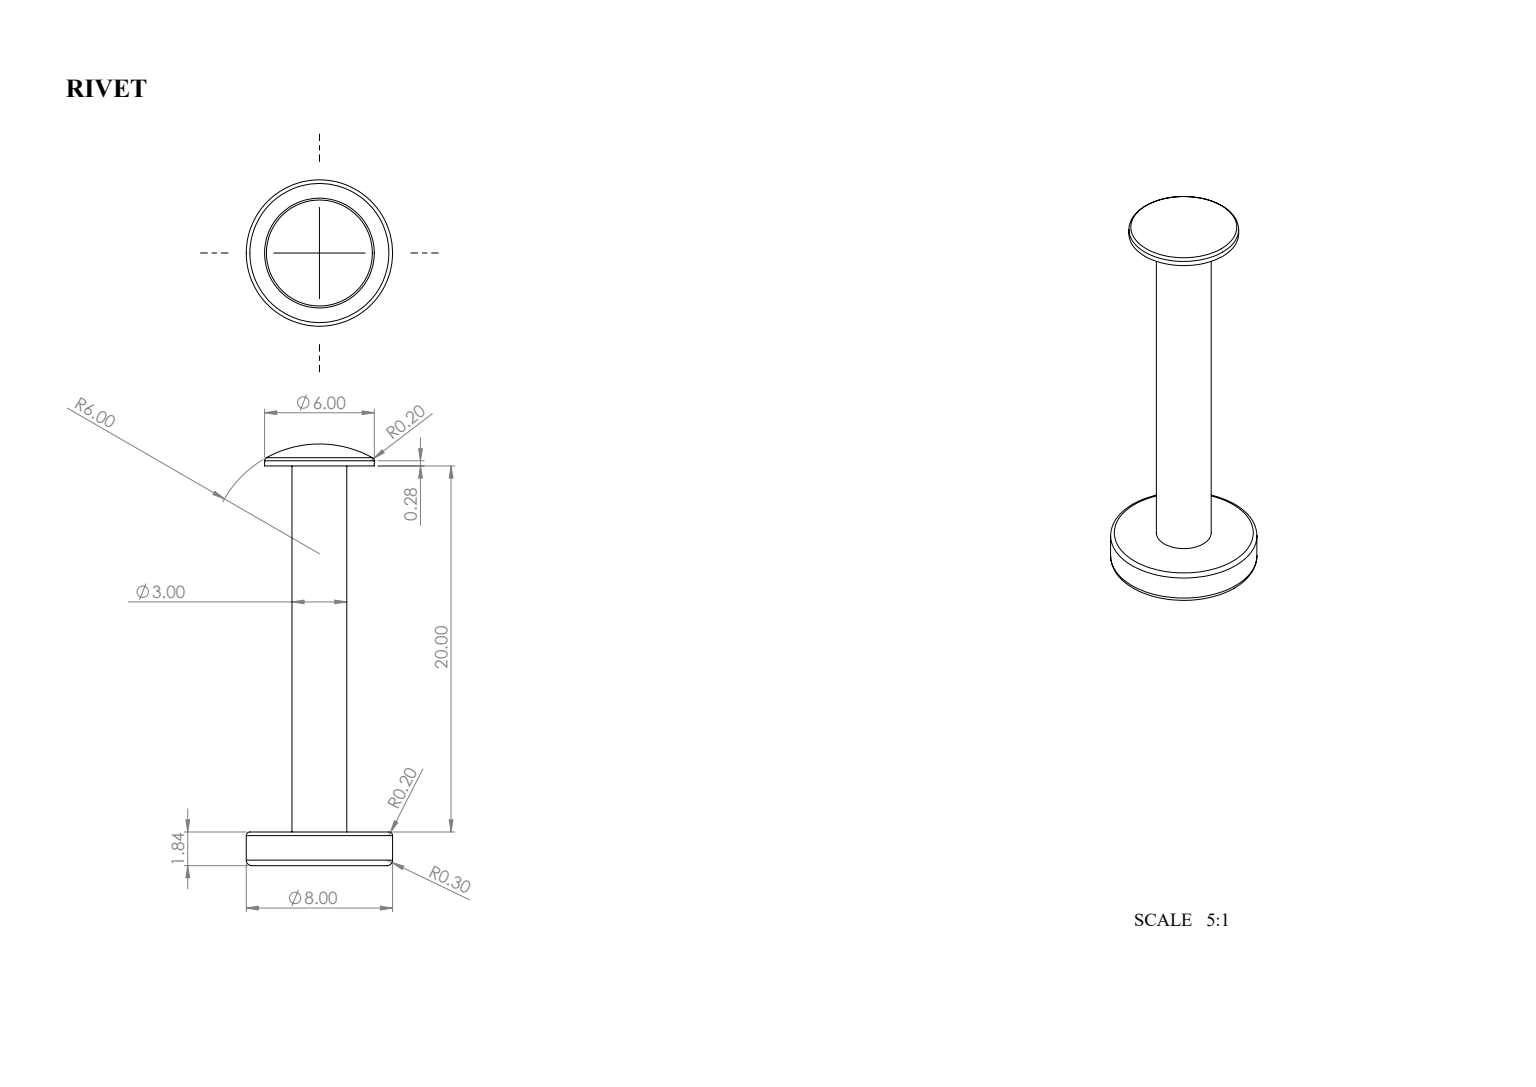
ISO-10303-21;
HEADER;
FILE_DESCRIPTION (('STEP AP214'),
    '1' );
FILE_NAME ('1.4 Rivet.step',
    '2026-10-07T05:30:18',
    ( '' ),
    ( '' ),
    'SwSTEP 2.0',
    'SolidWorks 2021',
    '' );
FILE_SCHEMA (( 'AUTOMOTIVE_DESIGN' ));
ENDSEC;

DATA;
#994=LINE ( 'NONE', #30968, #8060 ) ;
#1053=EDGE_CURVE ( 'NONE', #87334, #57215, #41639, .T. ) ;
#1123=FACE_OUTER_BOUND ( 'NONE', #83548, .T. ) ;
#1979=DIRECTION ( 'NONE',  ( 1.257568779154408793E-17, 1.000000000000000000, -0.000000000000000000 ) ) ;
#2099=EDGE_CURVE ( 'NONE', #84532, #89907, #23376, .T. ) ;
#2341=DIRECTION ( 'NONE',  ( 1.257568779154408793E-17, 1.000000000000000000, -0.000000000000000000 ) ) ;
#2551=DIRECTION ( 'NONE',  ( 1.224646799147353454E-16, -1.540077580099091832E-33, 1.000000000000000000 ) ) ;
#2715=VECTOR ( 'NONE', #9049, 1000.000000000000000 ) ;
#2831=CARTESIAN_POINT ( 'NONE',  ( -3.999999999999999112, 1.639999999999999014, 0.000000000000000000 ) ) ;
#2905=AXIS2_PLACEMENT_3D ( 'NONE', #26099, #87086, #58050 ) ;
#2964=CYLINDRICAL_SURFACE ( 'NONE', #23170, 3.000000000000000000 ) ;
#3145=CIRCLE ( 'NONE', #81349, 3.000000000000000000 ) ;
#3237=ORIENTED_EDGE ( 'NONE', *, *, #29922, .F. ) ;
#3507=ORIENTED_EDGE ( 'NONE', *, *, #71148, .T. ) ;
#3526=DIRECTION ( 'NONE',  ( 1.224646799147353207E-16, -1.540077580099091490E-33, 1.000000000000000000 ) ) ;
#3594=CARTESIAN_POINT ( 'NONE',  ( 2.781662917646512463E-16, 22.11937003968011695, 0.000000000000000000 ) ) ;
#3598=ORIENTED_EDGE ( 'NONE', *, *, #21717, .T. ) ;
#3600=AXIS2_PLACEMENT_3D ( 'NONE', #83921, #45930, #15451 ) ;
#3653=DIRECTION ( 'NONE',  ( -1.000000000000000000, 0.000000000000000000, 0.000000000000000000 ) ) ;
#3899=AXIS2_PLACEMENT_3D ( 'NONE', #71999, #3526, #32526 ) ;
#4516=UNCERTAINTY_MEASURE_WITH_UNIT (LENGTH_MEASURE( 1.000000000000000082E-05 ), #93288, 'distance_accuracy_value', 'NONE');
#4564=DIRECTION ( 'NONE',  ( 1.000000000000000000, 0.000000000000000000, 0.000000000000000000 ) ) ;
#4762=( LENGTH_UNIT ( ) NAMED_UNIT ( * ) SI_UNIT ( .MILLI., .METRE. ) );
#4915=ADVANCED_FACE ( 'NONE', ( #17323 ), #7942, .T. ) ;
#5067=ORIENTED_EDGE ( 'NONE', *, *, #61966, .F. ) ;
#5482=AXIS2_PLACEMENT_3D ( 'NONE', #73120, #20635, #81616 ) ;
#5598=ORIENTED_EDGE ( 'NONE', *, *, #25141, .F. ) ;
#5632=ORIENTED_EDGE ( 'NONE', *, *, #30715, .T. ) ;
#5880=ORIENTED_EDGE ( 'NONE', *, *, #27317, .T. ) ;
#6443=ORIENTED_EDGE ( 'NONE', *, *, #20709, .F. ) ;
#6533=( NAMED_UNIT ( * ) PLANE_ANGLE_UNIT ( ) SI_UNIT ( $, .RADIAN. ) );
#6537=EDGE_LOOP ( 'NONE', ( #7707, #54007, #79650, #25763 ) ) ;
#6599=CARTESIAN_POINT ( 'NONE',  ( 2.897438467171757030E-16, 23.03999999999999915, 0.000000000000000000 ) ) ;
#6634=ORIENTED_EDGE ( 'NONE', *, *, #41779, .F. ) ;
#6707=CARTESIAN_POINT ( 'NONE',  ( -3.999999999999999112, 23.03999999999999915, 0.000000000000000000 ) ) ;
#7105=AXIS2_PLACEMENT_3D ( 'NONE', #24931, #81354, #96380 ) ;
#7707=ORIENTED_EDGE ( 'NONE', *, *, #44953, .F. ) ;
#7942=TOROIDAL_SURFACE ( 'NONE', #95802, 3.699999999999999289, 0.2999999999999999889 ) ;
#8060=VECTOR ( 'NONE', #31455, 1000.000000000000000 ) ;
#8125=ORIENTED_EDGE ( 'NONE', *, *, #27988, .F. ) ;
#8242=DIRECTION ( 'NONE',  ( 1.257568779154408793E-17, 1.000000000000000000, -0.000000000000000000 ) ) ;
#8286=ORIENTED_EDGE ( 'NONE', *, *, #30815, .F. ) ;
#8311=CARTESIAN_POINT ( 'NONE',  ( 3.699999999999999289, -3.175805879500891925E-16, 0.000000000000000000 ) ) ;
#8356=DIRECTION ( 'NONE',  ( 1.000000000000000000, -1.257568779154408793E-17, 0.000000000000000000 ) ) ;
#8475=DIRECTION ( 'NONE',  ( -1.000000000000000000, 0.000000000000000000, 0.000000000000000000 ) ) ;
#8500=DIRECTION ( 'NONE',  ( 1.000000000000000000, -1.257568779154408793E-17, 0.000000000000000000 ) ) ;
#8588=CARTESIAN_POINT ( 'NONE',  ( 2.062412797813223616E-17, 1.639999999999999014, 0.000000000000000000 ) ) ;
#8590=DIRECTION ( 'NONE',  ( -1.224646799147353207E-16, 1.540077580099091490E-33, 1.000000000000000000 ) ) ;
#9030=ORIENTED_EDGE ( 'NONE', *, *, #22024, .T. ) ;
#9049=DIRECTION ( 'NONE',  ( 1.257568779154408793E-17, 1.000000000000000000, -0.000000000000000000 ) ) ;
#9309=SURFACE_STYLE_FILL_AREA ( #54796 ) ;
#9311=ADVANCED_FACE ( 'NONE', ( #80057 ), #12052, .T. ) ;
#9416=FACE_BOUND ( 'NONE', #37266, .T. ) ;
#9569=DIRECTION ( 'NONE',  ( -1.257568779154408793E-17, -1.000000000000000000, 0.000000000000000000 ) ) ;
#10064=ADVANCED_FACE ( 'NONE', ( #86449 ), #2964, .T. ) ;
#10245=EDGE_LOOP ( 'NONE', ( #5632, #31028 ) ) ;
#10593=FILL_AREA_STYLE_COLOUR ( '', #94402 ) ;
#10723=CIRCLE ( 'NONE', #42697, 3.799999999999998934 ) ;
#10781=FILL_AREA_STYLE ('',( #92794 ) ) ;
#10794=DIRECTION ( 'NONE',  ( 1.000000000000000000, -1.257568779154408793E-17, 0.000000000000000000 ) ) ;
#10894=DIRECTION ( 'NONE',  ( -1.000000000000000000, 1.257568779154408793E-17, 0.000000000000000000 ) ) ;
#11328=CIRCLE ( 'NONE', #49632, 5.999999999999998224 ) ;
#11443=CARTESIAN_POINT ( 'NONE',  ( 2.746530213673227803E-16, 21.83999999999999986, 0.000000000000000000 ) ) ;
#11508=CARTESIAN_POINT ( 'NONE',  ( -2.999999999999999556, 22.11937003968011695, 0.000000000000000000 ) ) ;
#11523=EDGE_CURVE ( 'NONE', #83267, #75676, #84199, .T. ) ;
#11994=VERTEX_POINT ( 'NONE', #72205 ) ;
#12052=CYLINDRICAL_SURFACE ( 'NONE', #51536, 3.999999999999999112 ) ;
#12174=ORIENTED_EDGE ( 'NONE', *, *, #68028, .F. ) ;
#12439=DIRECTION ( 'NONE',  ( 1.257568779154408793E-17, 1.000000000000000000, -0.000000000000000000 ) ) ;
#12451=CARTESIAN_POINT ( 'NONE',  ( 7.347880794884118750E-16, 17.03999999999999915, 0.000000000000000000 ) ) ;
#12652=VERTEX_POINT ( 'NONE', #39645 ) ;
#12891=AXIS2_PLACEMENT_3D ( 'NONE', #27041, #42546, #4564 ) ;
#13685=CARTESIAN_POINT ( 'NONE',  ( -3.799999999999998934, 1.839999999999999636, 0.000000000000000000 ) ) ;
#13872=EDGE_LOOP ( 'NONE', ( #80023, #45997, #3507, #3237 ) ) ;
#14332=CARTESIAN_POINT ( 'NONE',  ( 2.746530213673227803E-16, 21.83999999999999986, 0.000000000000000000 ) ) ;
#14481=UNCERTAINTY_MEASURE_WITH_UNIT (LENGTH_MEASURE( 1.000000000000000082E-05 ), #4762, 'distance_accuracy_value', 'NONE');
#14523=AXIS2_PLACEMENT_3D ( 'NONE', #8588, #9569, #70081 ) ;
#14902=DIRECTION ( 'NONE',  ( 1.257568779154408793E-17, 1.000000000000000000, -0.000000000000000000 ) ) ;
#15052=CARTESIAN_POINT ( 'NONE',  ( -1.499999999999998668, 1.840000000000001412, 0.000000000000000000 ) ) ;
#15404=EDGE_CURVE ( 'NONE', #57215, #87334, #18798, .T. ) ;
#15451=DIRECTION ( 'NONE',  ( -1.000000000000000000, 0.000000000000000000, 0.000000000000000000 ) ) ;
#15628=DIRECTION ( 'NONE',  ( 0.000000000000000000, -0.000000000000000000, -1.000000000000000000 ) ) ;
#15653=VERTEX_POINT ( 'NONE', #15052 ) ;
#15929=STYLED_ITEM ( 'NONE', ( #47796 ), #4915 ) ;
#16369=EDGE_CURVE ( 'NONE', #44561, #15653, #23678, .T. ) ;
#16487=ORIENTED_EDGE ( 'NONE', *, *, #71397, .T. ) ;
#16857=CARTESIAN_POINT ( 'NONE',  ( 2.313926553644105868E-17, 1.839999999999999636, 0.000000000000000000 ) ) ;
#17128=CIRCLE ( 'NONE', #21912, 3.000000000000000000 ) ;
#17130=ORIENTED_EDGE ( 'NONE', *, *, #2099, .F. ) ;
#17323=FACE_OUTER_BOUND ( 'NONE', #53241, .T. ) ;
#17492=DIRECTION ( 'NONE',  ( 1.257568779154408793E-17, 1.000000000000000000, -0.000000000000000000 ) ) ;
#17650=ORIENTED_EDGE ( 'NONE', *, *, #11523, .F. ) ;
#18398=ORIENTED_EDGE ( 'NONE', *, *, #82949, .T. ) ;
#18589=SURFACE_STYLE_USAGE ( .BOTH. , #71600 ) ;
#18679=( NAMED_UNIT ( * ) PLANE_ANGLE_UNIT ( ) SI_UNIT ( $, .RADIAN. ) );
#18798=CIRCLE ( 'NONE', #2905, 3.999999999999999112 ) ;
#19594=AXIS2_PLACEMENT_3D ( 'NONE', #63015, #2551, #39053 ) ;
#19664=CIRCLE ( 'NONE', #88330, 3.699999999999999289 ) ;
#19820=ORIENTED_EDGE ( 'NONE', *, *, #24624, .F. ) ;
#20445=CARTESIAN_POINT ( 'NONE',  ( 2.062412797813223616E-17, 1.639999999999999014, 0.000000000000000000 ) ) ;
#20635=DIRECTION ( 'NONE',  ( 0.000000000000000000, -0.000000000000000000, -1.000000000000000000 ) ) ;
#20709=EDGE_CURVE ( 'NONE', #89907, #69690, #91120, .T. ) ;
#20713=( GEOMETRIC_REPRESENTATION_CONTEXT ( 3 ) GLOBAL_UNCERTAINTY_ASSIGNED_CONTEXT ( ( #71206 ) ) GLOBAL_UNIT_ASSIGNED_CONTEXT ( ( #33757, #93792, #49275 ) ) REPRESENTATION_CONTEXT ( 'NONE', 'WORKASPACE' ) );
#20742=PRESENTATION_STYLE_ASSIGNMENT (( #78285 ) ) ;
#20764=CIRCLE ( 'NONE', #30309, 2.896551724137931494 ) ;
#20835=DIRECTION ( 'NONE',  ( -1.000000000000000000, 0.000000000000000000, 0.000000000000000000 ) ) ;
#21115=FACE_OUTER_BOUND ( 'NONE', #87748, .T. ) ;
#21186=ORIENTED_EDGE ( 'NONE', *, *, #61966, .T. ) ;
#21539=DIRECTION ( 'NONE',  ( 1.257568779154408793E-17, 1.000000000000000000, -0.000000000000000000 ) ) ;
#21717=EDGE_CURVE ( 'NONE', #44781, #46487, #11328, .T. ) ;
#21912=AXIS2_PLACEMENT_3D ( 'NONE', #3594, #57552, #56099 ) ;
#21942=LINE ( 'NONE', #52420, #54065 ) ;
#22024=EDGE_CURVE ( 'NONE', #46930, #46487, #86217, .T. ) ;
#22133=CARTESIAN_POINT ( 'NONE',  ( 2.800000000000000266, 22.11937003968011695, 0.000000000000000000 ) ) ;
#22137=CARTESIAN_POINT ( 'NONE',  ( -3.396451007058964006E-33, -2.700807354125587310E-16, 0.000000000000000000 ) ) ;
#22235=ORIENTED_EDGE ( 'NONE', *, *, #78802, .T. ) ;
#22388=DIRECTION ( 'NONE',  ( 1.257568779154408793E-17, 1.000000000000000000, -0.000000000000000000 ) ) ;
#22630=DIRECTION ( 'NONE',  ( -1.000000000000000000, 0.000000000000000000, 0.000000000000000000 ) ) ;
#22655=ORIENTED_EDGE ( 'NONE', *, *, #41779, .T. ) ;
#22759=ORIENTED_EDGE ( 'NONE', *, *, #56214, .T. ) ;
#23170=AXIS2_PLACEMENT_3D ( 'NONE', #77949, #1979, #8475 ) ;
#23376=LINE ( 'NONE', #38369, #94145 ) ;
#23678=CIRCLE ( 'NONE', #79537, 1.499999999999998668 ) ;
#23755=EDGE_LOOP ( 'NONE', ( #32187, #18398 ) ) ;
#24014=ORIENTED_EDGE ( 'NONE', *, *, #22024, .F. ) ;
#24324=( NAMED_UNIT ( * ) PLANE_ANGLE_UNIT ( ) SI_UNIT ( $, .RADIAN. ) );
#24336=FILL_AREA_STYLE_COLOUR ( '', #98967 ) ;
#24433=CARTESIAN_POINT ( 'NONE',  ( 7.347880794884118750E-16, 17.03999999999999915, 0.000000000000000000 ) ) ;
#24497=CARTESIAN_POINT ( 'NONE',  ( -2.896551724137927497, 22.29452073070357088, 0.000000000000000000 ) ) ;
#24624=EDGE_CURVE ( 'NONE', #57215, #34811, #44198, .T. ) ;
#24674=CIRCLE ( 'NONE', #61410, 0.2000000000000000944 ) ;
#24708=CARTESIAN_POINT ( 'NONE',  ( 3.772706337463130544E-18, 0.2999999999999981570, 0.000000000000000000 ) ) ;
#24931=CARTESIAN_POINT ( 'NONE',  ( -7.598395483715266452E-32, -2.710505431213761085E-16, 0.000000000000000000 ) ) ;
#25141=EDGE_CURVE ( 'NONE', #46930, #89907, #93033, .T. ) ;
#25327=TOROIDAL_SURFACE ( 'NONE', #82766, 3.799999999999998934, 0.2000000000000000111 ) ;
#25464=EDGE_CURVE ( 'NONE', #56371, #62932, #19664, .T. ) ;
#25535=DIRECTION ( 'NONE',  ( -1.000000000000000000, 0.000000000000000000, 0.000000000000000000 ) ) ;
#25540=EDGE_LOOP ( 'NONE', ( #67042, #60814, #9030 ) ) ;
#25576=DIRECTION ( 'NONE',  ( 1.000000000000000000, 0.000000000000000000, 1.224646799147350742E-16 ) ) ;
#25763=ORIENTED_EDGE ( 'NONE', *, *, #33913, .T. ) ;
#25811=FACE_OUTER_BOUND ( 'NONE', #51959, .T. ) ;
#26099=CARTESIAN_POINT ( 'NONE',  ( 3.772706337463130544E-18, 0.2999999999999981570, 0.000000000000000000 ) ) ;
#26995=CARTESIAN_POINT ( 'NONE',  ( -3.699999999999999289, -2.245204982926630245E-16, 4.714890176717308529E-16 ) ) ;
#27041=CARTESIAN_POINT ( 'NONE',  ( 2.781662917646512463E-16, 22.11937003968011695, 0.000000000000000000 ) ) ;
#27140=CARTESIAN_POINT ( 'NONE',  ( 3.772706337463130544E-18, 0.2999999999999981570, 0.000000000000000000 ) ) ;
#27242=( NAMED_UNIT ( * ) PLANE_ANGLE_UNIT ( ) SI_UNIT ( $, .RADIAN. ) );
#27317=EDGE_CURVE ( 'NONE', #98193, #84532, #3145, .T. ) ;
#27487=PRODUCT_DEFINITION_CONTEXT ( 'detailed design', #47424, 'design' ) ;
#27931=AXIS2_PLACEMENT_3D ( 'NONE', #67341, #59335, #50356 ) ;
#27940=FACE_OUTER_BOUND ( 'NONE', #25540, .T. ) ;
#27974=AXIS2_PLACEMENT_3D ( 'NONE', #68743, #46237, #77213 ) ;
#27988=EDGE_CURVE ( 'NONE', #44781, #46930, #20764, .T. ) ;
#28029=CARTESIAN_POINT ( 'NONE',  ( 4.428481664934704527E-16, 23.03999999999999915, 0.000000000000000000 ) ) ;
#28045=( LENGTH_UNIT ( ) NAMED_UNIT ( * ) SI_UNIT ( .MILLI., .METRE. ) );
#28235=ADVANCED_FACE ( 'NONE', ( #27940 ), #65443, .T. ) ;
#28251=CLOSED_SHELL ( 'NONE', ( #40089, #93361, #59049, #9311, #82063, #34808, #58866, #28235, #10064, #49984, #37767, #72656, #56477, #58568, #50063, #96661, #4915 ) ) ;
#28869=ORIENTED_EDGE ( 'NONE', *, *, #98825, .T. ) ;
#28911=DIRECTION ( 'NONE',  ( -1.000000000000000000, 0.000000000000000000, 0.000000000000000000 ) ) ;
#29922=EDGE_CURVE ( 'NONE', #12652, #52108, #10723, .T. ) ;
#30047=ORIENTED_EDGE ( 'NONE', *, *, #16369, .F. ) ;
#30276=EDGE_LOOP ( 'NONE', ( #12174, #65186 ) ) ;
#30309=AXIS2_PLACEMENT_3D ( 'NONE', #33463, #52660, #90654 ) ;
#30715=EDGE_CURVE ( 'NONE', #52108, #12652, #40920, .T. ) ;
#30720=CARTESIAN_POINT ( 'NONE',  ( 2.062412797813223616E-17, 1.639999999999999014, 0.000000000000000000 ) ) ;
#30815=EDGE_CURVE ( 'NONE', #11994, #34811, #53875, .T. ) ;
#30830=( GEOMETRIC_REPRESENTATION_CONTEXT ( 3 ) GLOBAL_UNCERTAINTY_ASSIGNED_CONTEXT ( ( #80431 ) ) GLOBAL_UNIT_ASSIGNED_CONTEXT ( ( #77688, #18679, #63172 ) ) REPRESENTATION_CONTEXT ( 'NONE', 'WORKASPACE' ) );
#30851=FACE_OUTER_BOUND ( 'NONE', #70276, .T. ) ;
#30968=CARTESIAN_POINT ( 'NONE',  ( 3.999999999999999112, 23.03999999999999915, 4.898587196589411843E-16 ) ) ;
#31028=ORIENTED_EDGE ( 'NONE', *, *, #29922, .T. ) ;
#31125=CARTESIAN_POINT ( 'NONE',  ( 3.000000000000000444, 22.11937003968011695, 3.673940397442059868E-16 ) ) ;
#31213=FACE_OUTER_BOUND ( 'NONE', #30276, .T. ) ;
#31347=DIRECTION ( 'NONE',  ( -1.000000000000000000, 0.000000000000000000, 0.000000000000000000 ) ) ;
#31455=DIRECTION ( 'NONE',  ( 1.257568779154408793E-17, 1.000000000000000000, -0.000000000000000000 ) ) ;
#31585=PLANE ( 'NONE',  #42803 ) ;
#31625=ORIENTED_EDGE ( 'NONE', *, *, #20709, .T. ) ;
#31773=DIRECTION ( 'NONE',  ( -1.000000000000000000, 0.000000000000000000, 0.000000000000000000 ) ) ;
#31791=SURFACE_SIDE_STYLE ('',( #72252 ) ) ;
#31889=MECHANICAL_DESIGN_GEOMETRIC_PRESENTATION_REPRESENTATION('',(#15929),#20713);
#31941=CARTESIAN_POINT ( 'NONE',  ( 2.896551724137929273, 22.29452073070357088, 3.547252797530261487E-16 ) ) ;
#32187=ORIENTED_EDGE ( 'NONE', *, *, #11523, .T. ) ;
#32234=ADVANCED_BREP_SHAPE_REPRESENTATION ( '', ( #74465, #27931 ), #93381 ) ;
#32376=DIRECTION ( 'NONE',  ( -1.224646799147353207E-16, 1.540077580099091490E-33, 1.000000000000000000 ) ) ;
#32526=DIRECTION ( 'NONE',  ( 1.000000000000000000, 0.000000000000000000, -1.224646799147353207E-16 ) ) ;
#32678=SURFACE_SIDE_STYLE ('',( #62682 ) ) ;
#32727=ORIENTED_EDGE ( 'NONE', *, *, #67690, .F. ) ;
#32777=( NAMED_UNIT ( * ) SI_UNIT ( $, .STERADIAN. ) SOLID_ANGLE_UNIT ( ) );
#33015=ORIENTED_EDGE ( 'NONE', *, *, #44953, .T. ) ;
#33463=CARTESIAN_POINT ( 'NONE',  ( 8.008672916919360803E-16, 22.29452073070357088, 0.000000000000000000 ) ) ;
#33702=EDGE_LOOP ( 'NONE', ( #81537, #3598, #24014 ) ) ;
#33757=( LENGTH_UNIT ( ) NAMED_UNIT ( * ) SI_UNIT ( .MILLI., .METRE. ) );
#33913=EDGE_CURVE ( 'NONE', #34811, #11994, #35252, .T. ) ;
#33951=DIRECTION ( 'NONE',  ( 0.000000000000000000, 0.000000000000000000, 1.000000000000000000 ) ) ;
#34142=DIRECTION ( 'NONE',  ( 1.257568779154408793E-17, 1.000000000000000000, -0.000000000000000000 ) ) ;
#34741=SHAPE_DEFINITION_REPRESENTATION ( #83359, #57512 ) ;
#34808=ADVANCED_FACE ( 'NONE', ( #25811 ), #61823, .T. ) ;
#34811=VERTEX_POINT ( 'NONE', #2831 ) ;
#35252=CIRCLE ( 'NONE', #14523, 3.999999999999999112 ) ;
#36064=EDGE_LOOP ( 'NONE', ( #22235, #22759, #17650, #40755 ) ) ;
#37112=DIRECTION ( 'NONE',  ( 1.257568779154408793E-17, 1.000000000000000000, -0.000000000000000000 ) ) ;
#37266=EDGE_LOOP ( 'NONE', ( #95845, #30047 ) ) ;
#37767=ADVANCED_FACE ( 'NONE', ( #21115 ), #83091, .T. ) ;
#37790=AXIS2_PLACEMENT_3D ( 'NONE', #65434, #12439, #56476 ) ;
#38369=CARTESIAN_POINT ( 'NONE',  ( -2.999999999999999556, 23.03999999999999915, 0.000000000000000000 ) ) ;
#39053=DIRECTION ( 'NONE',  ( 1.000000000000000000, 0.000000000000000000, -1.224646799147353207E-16 ) ) ;
#39185=DIRECTION ( 'NONE',  ( 1.000000000000000000, -1.257568779154408485E-17, 0.000000000000000000 ) ) ;
#39204=TOROIDAL_SURFACE ( 'NONE', #72711, 3.799999999999998934, 0.2000000000000000111 ) ;
#39236=FACE_OUTER_BOUND ( 'NONE', #13872, .T. ) ;
#39430=DIRECTION ( 'NONE',  ( 0.000000000000000000, 0.000000000000000000, 1.000000000000000000 ) ) ;
#39555=CARTESIAN_POINT ( 'NONE',  ( 2.746530213673227803E-16, 21.83999999999999986, 0.000000000000000000 ) ) ;
#39645=CARTESIAN_POINT ( 'NONE',  ( 3.799999999999998934, 1.839999999999999636, 4.776122516674677286E-16 ) ) ;
#40087=DIRECTION ( 'NONE',  ( 1.000000000000000000, -1.257568779154408793E-17, 0.000000000000000000 ) ) ;
#40089=ADVANCED_FACE ( 'NONE', ( #56665 ), #86742, .T. ) ;
#40494=STYLED_ITEM ( 'NONE', ( #69711 ), #40089 ) ;
#40755=ORIENTED_EDGE ( 'NONE', *, *, #71397, .F. ) ;
#40920=CIRCLE ( 'NONE', #37790, 3.799999999999998934 ) ;
#40967=AXIS2_PLACEMENT_3D ( 'NONE', #87377, #70421, #10894 ) ;
#40975=DIRECTION ( 'NONE',  ( -1.257568779154408793E-17, -1.000000000000000000, 0.000000000000000000 ) ) ;
#41107=FILL_AREA_STYLE ('',( #10593 ) ) ;
#41195=DIRECTION ( 'NONE',  ( 1.000000000000000000, -1.355252715606880851E-17, 0.000000000000000000 ) ) ;
#41278=CARTESIAN_POINT ( 'NONE',  ( -1.499999999999998890, 21.83999999999999986, 0.000000000000000000 ) ) ;
#41639=CIRCLE ( 'NONE', #84738, 3.999999999999999112 ) ;
#41779=EDGE_CURVE ( 'NONE', #98193, #69690, #59955, .T. ) ;
#41962=DIRECTION ( 'NONE',  ( -1.000000000000000000, 0.000000000000000000, 0.000000000000000000 ) ) ;
#42329=APPLICATION_CONTEXT ( 'automotive_design' ) ;
#42546=DIRECTION ( 'NONE',  ( -1.257568779154408793E-17, -1.000000000000000000, 0.000000000000000000 ) ) ;
#42584=ORIENTED_EDGE ( 'NONE', *, *, #15404, .T. ) ;
#42697=AXIS2_PLACEMENT_3D ( 'NONE', #16857, #14902, #31347 ) ;
#42803=AXIS2_PLACEMENT_3D ( 'NONE', #22137, #52620, #40087 ) ;
#43605=AXIS2_PLACEMENT_3D ( 'NONE', #24708, #92696, #56187 ) ;
#44198=LINE ( 'NONE', #6707, #70716 ) ;
#44561=VERTEX_POINT ( 'NONE', #61565 ) ;
#44781=VERTEX_POINT ( 'NONE', #31941 ) ;
#44953=EDGE_CURVE ( 'NONE', #87334, #11994, #994, .T. ) ;
#45086=DIRECTION ( 'NONE',  ( -1.000000000000000000, 0.000000000000000000, 0.000000000000000000 ) ) ;
#45793=AXIS2_PLACEMENT_3D ( 'NONE', #70828, #2341, #92331 ) ;
#45930=DIRECTION ( 'NONE',  ( 1.257568779154408793E-17, 1.000000000000000000, -0.000000000000000000 ) ) ;
#45997=ORIENTED_EDGE ( 'NONE', *, *, #33913, .F. ) ;
#46237=DIRECTION ( 'NONE',  ( -1.257568779154408793E-17, -1.000000000000000000, 0.000000000000000000 ) ) ;
#46451=CARTESIAN_POINT ( 'NONE',  ( 2.897438467171757030E-16, 23.03999999999999915, 0.000000000000000000 ) ) ;
#46487=VERTEX_POINT ( 'NONE', #28029 ) ;
#46930=VERTEX_POINT ( 'NONE', #24497 ) ;
#46997=CIRCLE ( 'NONE', #3899, 0.2999999999999999334 ) ;
#47055=COLOUR_RGB ( '', 0.09019608, 0.27058824, 0.51372549) ;
#47424=APPLICATION_CONTEXT ( 'automotive_design' ) ;
#47692=SURFACE_STYLE_USAGE ( .BOTH. , #32678 ) ;
#47796=PRESENTATION_STYLE_ASSIGNMENT (( #48778 ) ) ;
#48087=ORIENTED_EDGE ( 'NONE', *, *, #25464, .F. ) ;
#48778=SURFACE_STYLE_USAGE ( .BOTH. , #71305 ) ;
#48898=PRODUCT_DEFINITION ( 'UNKNOWN', '', #75905, #27487 ) ;
#49074=AXIS2_PLACEMENT_3D ( 'NONE', #39555, #85535, #25535 ) ;
#49082=PRESENTATION_STYLE_ASSIGNMENT (( #18589 ) ) ;
#49096=ORIENTED_EDGE ( 'NONE', *, *, #94809, .T. ) ;
#49275=( NAMED_UNIT ( * ) SI_UNIT ( $, .STERADIAN. ) SOLID_ANGLE_UNIT ( ) );
#49632=AXIS2_PLACEMENT_3D ( 'NONE', #92394, #32376, #70894 ) ;
#49984=ADVANCED_FACE ( 'NONE', ( #61229, #31213 ), #61709, .T. ) ;
#50054=DIRECTION ( 'NONE',  ( -1.000000000000000000, 0.000000000000000000, 0.000000000000000000 ) ) ;
#50063=ADVANCED_FACE ( 'NONE', ( #39236 ), #39204, .T. ) ;
#50158=ORIENTED_EDGE ( 'NONE', *, *, #97928, .F. ) ;
#50257=MECHANICAL_DESIGN_GEOMETRIC_PRESENTATION_REPRESENTATION('',(#67848),#56702);
#50289=DIRECTION ( 'NONE',  ( 1.257568779154408793E-17, 1.000000000000000000, -0.000000000000000000 ) ) ;
#50356=DIRECTION ( 'NONE',  ( 1.000000000000000000, 0.000000000000000000, 0.000000000000000000 ) ) ;
#50723=AXIS2_PLACEMENT_3D ( 'NONE', #74031, #97559, #81534 ) ;
#50801=DIRECTION ( 'NONE',  ( -1.000000000000000000, 1.257568779154408793E-17, 0.000000000000000000 ) ) ;
#50934=DIRECTION ( 'NONE',  ( -1.257568779154408793E-17, -1.000000000000000000, 0.000000000000000000 ) ) ;
#51304=STYLED_ITEM ( 'NONE', ( #49082 ), #74465 ) ;
#51536=AXIS2_PLACEMENT_3D ( 'NONE', #73528, #21539, #50054 ) ;
#51930=CARTESIAN_POINT ( 'NONE',  ( 2.313926553644108641E-17, 1.840000000000001412, 0.000000000000000000 ) ) ;
#51959=EDGE_LOOP ( 'NONE', ( #85832, #22655, #66185, #17130 ) ) ;
#52108=VERTEX_POINT ( 'NONE', #13685 ) ;
#52420=CARTESIAN_POINT ( 'NONE',  ( -1.499999999999998668, 23.03999999999999915, 0.000000000000000000 ) ) ;
#52620=DIRECTION ( 'NONE',  ( -1.257568779154408793E-17, -1.000000000000000000, 0.000000000000000000 ) ) ;
#52660=DIRECTION ( 'NONE',  ( 1.257568779154408793E-17, 1.000000000000000000, -0.000000000000000000 ) ) ;
#52738=DIRECTION ( 'NONE',  ( -1.000000000000000000, 1.257568779154408793E-17, 0.000000000000000000 ) ) ;
#52933=FACE_OUTER_BOUND ( 'NONE', #33702, .T. ) ;
#53241=EDGE_LOOP ( 'NONE', ( #50158, #75044, #49096, #48087 ) ) ;
#53253=MECHANICAL_DESIGN_GEOMETRIC_PRESENTATION_REPRESENTATION('',(#40494),#30830);
#53413=CYLINDRICAL_SURFACE ( 'NONE', #3600, 1.499999999999998890 ) ;
#53439=DIRECTION ( 'NONE',  ( 1.257568779154408793E-17, 1.000000000000000000, -0.000000000000000000 ) ) ;
#53796=AXIS2_PLACEMENT_3D ( 'NONE', #46451, #75471, #76944 ) ;
#53875=CIRCLE ( 'NONE', #72973, 3.999999999999999112 ) ;
#53953=FACE_OUTER_BOUND ( 'NONE', #6537, .T. ) ;
#54007=ORIENTED_EDGE ( 'NONE', *, *, #1053, .T. ) ;
#54065=VECTOR ( 'NONE', #98447, 1000.000000000000000 ) ;
#54109=UNCERTAINTY_MEASURE_WITH_UNIT (LENGTH_MEASURE( 1.000000000000000082E-05 ), #28045, 'distance_accuracy_value', 'NONE');
#54392=AXIS2_PLACEMENT_3D ( 'NONE', #72125, #73597, #3653 ) ;
#54445=CARTESIAN_POINT ( 'NONE',  ( 1.499999999999999556, 21.83999999999999986, 1.836970198721029194E-16 ) ) ;
#54796=FILL_AREA_STYLE ('',( #24336 ) ) ;
#55179=FILL_AREA_STYLE_COLOUR ( '', #83591 ) ;
#55907=FACE_OUTER_BOUND ( 'NONE', #10245, .T. ) ;
#56099=DIRECTION ( 'NONE',  ( 1.000000000000000000, 0.000000000000000000, 0.000000000000000000 ) ) ;
#56187=DIRECTION ( 'NONE',  ( 1.000000000000000000, -1.257568779154408793E-17, 0.000000000000000000 ) ) ;
#56214=EDGE_CURVE ( 'NONE', #44561, #75676, #85048, .T. ) ;
#56371=VERTEX_POINT ( 'NONE', #26995 ) ;
#56476=DIRECTION ( 'NONE',  ( -1.000000000000000000, 0.000000000000000000, 0.000000000000000000 ) ) ;
#56477=ADVANCED_FACE ( 'NONE', ( #53953 ), #90954, .T. ) ;
#56665=FACE_OUTER_BOUND ( 'NONE', #73673, .T. ) ;
#56702=( GEOMETRIC_REPRESENTATION_CONTEXT ( 3 ) GLOBAL_UNCERTAINTY_ASSIGNED_CONTEXT ( ( #14481 ) ) GLOBAL_UNIT_ASSIGNED_CONTEXT ( ( #4762, #27242, #80749 ) ) REPRESENTATION_CONTEXT ( 'NONE', 'WORKASPACE' ) );
#57215=VERTEX_POINT ( 'NONE', #68695 ) ;
#57512=SHAPE_REPRESENTATION ( '1.4 Rivet', ( #27931 ), #93381 ) ;
#57552=DIRECTION ( 'NONE',  ( -1.257568779154408793E-17, -1.000000000000000000, 0.000000000000000000 ) ) ;
#58050=DIRECTION ( 'NONE',  ( 1.000000000000000000, -1.355252715606880851E-17, 0.000000000000000000 ) ) ;
#58424=DIRECTION ( 'NONE',  ( 1.257568779154408793E-17, 1.000000000000000000, -0.000000000000000000 ) ) ;
#58469=ORIENTED_EDGE ( 'NONE', *, *, #25141, .T. ) ;
#58568=ADVANCED_FACE ( 'NONE', ( #1123 ), #31585, .T. ) ;
#58729=SHAPE_REPRESENTATION_RELATIONSHIP ( 'NONE' , 'NONE' ,  #57512, #32234 ) ;
#58866=ADVANCED_FACE ( 'NONE', ( #52933 ), #75937, .T. ) ;
#58935=CARTESIAN_POINT ( 'NONE',  ( -3.799999999999998934, 1.639999999999999014, 0.000000000000000000 ) ) ;
#59049=ADVANCED_FACE ( 'NONE', ( #59274 ), #25327, .T. ) ;
#59065=EDGE_LOOP ( 'NONE', ( #42584, #33015, #61264, #19820 ) ) ;
#59274=FACE_OUTER_BOUND ( 'NONE', #66174, .T. ) ;
#59335=DIRECTION ( 'NONE',  ( 0.000000000000000000, 0.000000000000000000, 1.000000000000000000 ) ) ;
#59463=CARTESIAN_POINT ( 'NONE',  ( 3.000000000000000444, 23.03999999999999915, 3.673940397442059868E-16 ) ) ;
#59955=LINE ( 'NONE', #59463, #80751 ) ;
#60814=ORIENTED_EDGE ( 'NONE', *, *, #27988, .T. ) ;
#61229=FACE_BOUND ( 'NONE', #23755, .T. ) ;
#61264=ORIENTED_EDGE ( 'NONE', *, *, #30815, .T. ) ;
#61410=AXIS2_PLACEMENT_3D ( 'NONE', #87044, #8590, #25576 ) ;
#61565=CARTESIAN_POINT ( 'NONE',  ( 1.499999999999998668, 1.840000000000001412, 1.836970198721028701E-16 ) ) ;
#61709=PLANE ( 'NONE',  #27974 ) ;
#61823=CYLINDRICAL_SURFACE ( 'NONE', #45793, 3.000000000000000000 ) ;
#61966=EDGE_CURVE ( 'NONE', #44781, #69690, #79977, .T. ) ;
#62299=CARTESIAN_POINT ( 'NONE',  ( 3.772706337463130544E-18, 0.2999999999999981570, 0.000000000000000000 ) ) ;
#62682=SURFACE_STYLE_FILL_AREA ( #70700 ) ;
#62904=ORIENTED_EDGE ( 'NONE', *, *, #16369, .T. ) ;
#62913=CIRCLE ( 'NONE', #5482, 0.2999999999999999334 ) ;
#62932=VERTEX_POINT ( 'NONE', #8311 ) ;
#63015=CARTESIAN_POINT ( 'NONE',  ( -2.799999999999999378, 22.11937003968011695, 3.429011037612589769E-16 ) ) ;
#63172=( NAMED_UNIT ( * ) SI_UNIT ( $, .STERADIAN. ) SOLID_ANGLE_UNIT ( ) );
#63692=CIRCLE ( 'NONE', #78055, 0.2000000000000000944 ) ;
#64234=CARTESIAN_POINT ( 'NONE',  ( 8.008672916919360803E-16, 22.29452073070357088, 0.000000000000000000 ) ) ;
#64395=TOROIDAL_SURFACE ( 'NONE', #90172, 2.799999999999999822, 0.2000000000000000111 ) ;
#64905=AXIS2_PLACEMENT_3D ( 'NONE', #6599, #37112, #45086 ) ;
#65186=ORIENTED_EDGE ( 'NONE', *, *, #27317, .F. ) ;
#65192=AXIS2_PLACEMENT_3D ( 'NONE', #24433, #39430, #68940 ) ;
#65255=ORIENTED_EDGE ( 'NONE', *, *, #95402, .T. ) ;
#65434=CARTESIAN_POINT ( 'NONE',  ( 2.313926553644105868E-17, 1.839999999999999636, 0.000000000000000000 ) ) ;
#65443=SPHERICAL_SURFACE ( 'NONE', #76648, 5.999999999999998224 ) ;
#65474=CARTESIAN_POINT ( 'NONE',  ( 3.000000000000000444, 21.83999999999999986, 3.673940397442059868E-16 ) ) ;
#65952=AXIS2_PLACEMENT_3D ( 'NONE', #14332, #91800, #31773 ) ;
#66056=AXIS2_PLACEMENT_3D ( 'NONE', #78956, #40975, #8500 ) ;
#66174=EDGE_LOOP ( 'NONE', ( #8286, #65255, #73272, #78134 ) ) ;
#66185=ORIENTED_EDGE ( 'NONE', *, *, #67690, .T. ) ;
#66473=CIRCLE ( 'NONE', #87238, 2.896551724137931494 ) ;
#66639=CIRCLE ( 'NONE', #50723, 3.000000000000000000 ) ;
#67042=ORIENTED_EDGE ( 'NONE', *, *, #21717, .F. ) ;
#67341=CARTESIAN_POINT ( 'NONE',  ( 0.000000000000000000, 0.000000000000000000, 0.000000000000000000 ) ) ;
#67690=EDGE_CURVE ( 'NONE', #69690, #89907, #17128, .T. ) ;
#67848=STYLED_ITEM ( 'NONE', ( #20742 ), #32234 ) ;
#68028=EDGE_CURVE ( 'NONE', #84532, #98193, #66639, .T. ) ;
#68186=ORIENTED_EDGE ( 'NONE', *, *, #98825, .F. ) ;
#68692=DIRECTION ( 'NONE',  ( -1.257568779154408793E-17, -1.000000000000000000, 0.000000000000000000 ) ) ;
#68694=DIRECTION ( 'NONE',  ( 1.257568779154408793E-17, 1.000000000000000000, -0.000000000000000000 ) ) ;
#68695=CARTESIAN_POINT ( 'NONE',  ( -3.999999999999999112, 0.2999999999999982125, 0.000000000000000000 ) ) ;
#68743=CARTESIAN_POINT ( 'NONE',  ( -1.499999999999998890, 21.83999999999999986, 0.000000000000000000 ) ) ;
#68869=DIRECTION ( 'NONE',  ( -1.257568779154408793E-17, -1.000000000000000000, 0.000000000000000000 ) ) ;
#68940=DIRECTION ( 'NONE',  ( -1.000000000000000000, 0.000000000000000000, 0.000000000000000000 ) ) ;
#69690=VERTEX_POINT ( 'NONE', #31125 ) ;
#69711=PRESENTATION_STYLE_ASSIGNMENT (( #47692 ) ) ;
#70081=DIRECTION ( 'NONE',  ( -1.000000000000000000, 0.000000000000000000, 0.000000000000000000 ) ) ;
#70276=EDGE_LOOP ( 'NONE', ( #5598, #8125, #21186, #6443 ) ) ;
#70344=CARTESIAN_POINT ( 'NONE',  ( 2.781662917646512463E-16, 22.11937003968011695, 0.000000000000000000 ) ) ;
#70421=DIRECTION ( 'NONE',  ( 1.257568779154408793E-17, 1.000000000000000000, -0.000000000000000000 ) ) ;
#70424=AXIS2_PLACEMENT_3D ( 'NONE', #22133, #15628, #22630 ) ;
#70515=MECHANICAL_DESIGN_GEOMETRIC_PRESENTATION_REPRESENTATION('',(#51304),#76854);
#70700=FILL_AREA_STYLE ('',( #55179 ) ) ;
#70716=VECTOR ( 'NONE', #68694, 1000.000000000000000 ) ;
#70768=CIRCLE ( 'NONE', #65952, 1.499999999999999112 ) ;
#70818=DIRECTION ( 'NONE',  ( -1.257568779154408793E-17, -1.000000000000000000, 0.000000000000000000 ) ) ;
#70828=CARTESIAN_POINT ( 'NONE',  ( 2.897438467171757030E-16, 23.03999999999999915, 0.000000000000000000 ) ) ;
#70894=DIRECTION ( 'NONE',  ( 1.000000000000000000, 0.000000000000000000, 1.224646799147353207E-16 ) ) ;
#71148=EDGE_CURVE ( 'NONE', #34811, #52108, #63692, .T. ) ;
#71206=UNCERTAINTY_MEASURE_WITH_UNIT (LENGTH_MEASURE( 1.000000000000000082E-05 ), #33757, 'distance_accuracy_value', 'NONE');
#71305=SURFACE_SIDE_STYLE ('',( #9309 ) ) ;
#71397=EDGE_CURVE ( 'NONE', #15653, #83267, #21942, .T. ) ;
#71600=SURFACE_SIDE_STYLE ('',( #94575 ) ) ;
#71999=CARTESIAN_POINT ( 'NONE',  ( -3.699999999999999289, 0.2999999999999982125, 4.531193156845205215E-16 ) ) ;
#72125=CARTESIAN_POINT ( 'NONE',  ( 2.313926553644108641E-17, 1.840000000000001412, 0.000000000000000000 ) ) ;
#72205=CARTESIAN_POINT ( 'NONE',  ( 3.999999999999999112, 1.639999999999999014, 4.898587196589411843E-16 ) ) ;
#72252=SURFACE_STYLE_FILL_AREA ( #10781 ) ;
#72656=ADVANCED_FACE ( 'NONE', ( #55907, #9416 ), #94876, .T. ) ;
#72711=AXIS2_PLACEMENT_3D ( 'NONE', #30720, #8242, #52738 ) ;
#72973=AXIS2_PLACEMENT_3D ( 'NONE', #20445, #50934, #73928 ) ;
#73120=CARTESIAN_POINT ( 'NONE',  ( 3.699999999999999289, 0.2999999999999981570, 0.000000000000000000 ) ) ;
#73272=ORIENTED_EDGE ( 'NONE', *, *, #30715, .F. ) ;
#73328=CARTESIAN_POINT ( 'NONE',  ( 7.347880794884118750E-16, 17.03999999999999915, 0.000000000000000000 ) ) ;
#73528=CARTESIAN_POINT ( 'NONE',  ( 2.897438467171757030E-16, 23.03999999999999915, 0.000000000000000000 ) ) ;
#73597=DIRECTION ( 'NONE',  ( 1.257568779154408793E-17, 1.000000000000000000, -0.000000000000000000 ) ) ;
#73673=EDGE_LOOP ( 'NONE', ( #82554, #76758, #68186, #79117 ) ) ;
#73876=ORIENTED_EDGE ( 'NONE', *, *, #88262, .F. ) ;
#73928=DIRECTION ( 'NONE',  ( -1.000000000000000000, 0.000000000000000000, 0.000000000000000000 ) ) ;
#74031=CARTESIAN_POINT ( 'NONE',  ( 2.746530213673227803E-16, 21.83999999999999986, 0.000000000000000000 ) ) ;
#74047=TOROIDAL_SURFACE ( 'NONE', #66056, 2.799999999999999822, 0.2000000000000000111 ) ;
#74200=DIRECTION ( 'NONE',  ( 1.257568779154408793E-17, 1.000000000000000000, -0.000000000000000000 ) ) ;
#74465=MANIFOLD_SOLID_BREP ( 'Fillet2', #28251 ) ;
#75044=ORIENTED_EDGE ( 'NONE', *, *, #1053, .F. ) ;
#75471=DIRECTION ( 'NONE',  ( 1.257568779154408793E-17, 1.000000000000000000, -0.000000000000000000 ) ) ;
#75676=VERTEX_POINT ( 'NONE', #54445 ) ;
#75761=CIRCLE ( 'NONE', #7105, 3.699999999999999289 ) ;
#75905=PRODUCT_DEFINITION_FORMATION_WITH_SPECIFIED_SOURCE ( 'ANY', '', #98572, .NOT_KNOWN. ) ;
#75925=FACE_OUTER_BOUND ( 'NONE', #36064, .T. ) ;
#75937=SPHERICAL_SURFACE ( 'NONE', #65192, 5.999999999999998224 ) ;
#76181=CARTESIAN_POINT ( 'NONE',  ( 3.999999999999999112, 0.2999999999999981570, 4.898587196589411843E-16 ) ) ;
#76648=AXIS2_PLACEMENT_3D ( 'NONE', #12451, #33951, #88947 ) ;
#76758=ORIENTED_EDGE ( 'NONE', *, *, #97928, .T. ) ;
#76854=( GEOMETRIC_REPRESENTATION_CONTEXT ( 3 ) GLOBAL_UNCERTAINTY_ASSIGNED_CONTEXT ( ( #54109 ) ) GLOBAL_UNIT_ASSIGNED_CONTEXT ( ( #28045, #6533, #83030 ) ) REPRESENTATION_CONTEXT ( 'NONE', 'WORKASPACE' ) );
#76944=DIRECTION ( 'NONE',  ( -1.000000000000000000, 0.000000000000000000, 0.000000000000000000 ) ) ;
#77213=DIRECTION ( 'NONE',  ( 1.000000000000000000, -1.257568779154408793E-17, 0.000000000000000000 ) ) ;
#77471=FACE_OUTER_BOUND ( 'NONE', #98772, .T. ) ;
#77531=CARTESIAN_POINT ( 'NONE',  ( 1.499999999999999112, 23.03999999999999915, 1.836970198721028701E-16 ) ) ;
#77688=( LENGTH_UNIT ( ) NAMED_UNIT ( * ) SI_UNIT ( .MILLI., .METRE. ) );
#77949=CARTESIAN_POINT ( 'NONE',  ( 2.897438467171757030E-16, 23.03999999999999915, 0.000000000000000000 ) ) ;
#78055=AXIS2_PLACEMENT_3D ( 'NONE', #58935, #89435, #97951 ) ;
#78134=ORIENTED_EDGE ( 'NONE', *, *, #71148, .F. ) ;
#78285=SURFACE_STYLE_USAGE ( .BOTH. , #31791 ) ;
#78802=EDGE_CURVE ( 'NONE', #15653, #44561, #97540, .T. ) ;
#78956=CARTESIAN_POINT ( 'NONE',  ( 2.781662917646512463E-16, 22.11937003968011695, 0.000000000000000000 ) ) ;
#79117=ORIENTED_EDGE ( 'NONE', *, *, #94809, .F. ) ;
#79537=AXIS2_PLACEMENT_3D ( 'NONE', #51930, #58424, #28911 ) ;
#79650=ORIENTED_EDGE ( 'NONE', *, *, #24624, .T. ) ;
#79977=CIRCLE ( 'NONE', #70424, 0.2000000000000000944 ) ;
#80023=ORIENTED_EDGE ( 'NONE', *, *, #95402, .F. ) ;
#80057=FACE_OUTER_BOUND ( 'NONE', #59065, .T. ) ;
#80431=UNCERTAINTY_MEASURE_WITH_UNIT (LENGTH_MEASURE( 1.000000000000000082E-05 ), #77688, 'distance_accuracy_value', 'NONE');
#80749=( NAMED_UNIT ( * ) SI_UNIT ( $, .STERADIAN. ) SOLID_ANGLE_UNIT ( ) );
#80751=VECTOR ( 'NONE', #53439, 1000.000000000000000 ) ;
#81349=AXIS2_PLACEMENT_3D ( 'NONE', #11443, #17492, #41962 ) ;
#81354=DIRECTION ( 'NONE',  ( -1.257568779154408793E-17, -1.000000000000000000, 0.000000000000000000 ) ) ;
#81534=DIRECTION ( 'NONE',  ( -1.000000000000000000, 0.000000000000000000, 0.000000000000000000 ) ) ;
#81537=ORIENTED_EDGE ( 'NONE', *, *, #88262, .T. ) ;
#81616=DIRECTION ( 'NONE',  ( -1.000000000000000000, 0.000000000000000000, 0.000000000000000000 ) ) ;
#82063=ADVANCED_FACE ( 'NONE', ( #75925 ), #53413, .T. ) ;
#82554=ORIENTED_EDGE ( 'NONE', *, *, #15404, .F. ) ;
#82766=AXIS2_PLACEMENT_3D ( 'NONE', #89288, #50289, #50801 ) ;
#82949=EDGE_CURVE ( 'NONE', #75676, #83267, #70768, .T. ) ;
#83030=( NAMED_UNIT ( * ) SI_UNIT ( $, .STERADIAN. ) SOLID_ANGLE_UNIT ( ) );
#83091=CYLINDRICAL_SURFACE ( 'NONE', #64905, 1.499999999999998890 ) ;
#83267=VERTEX_POINT ( 'NONE', #41278 ) ;
#83359=PRODUCT_DEFINITION_SHAPE ( 'NONE', 'NONE',  #48898 ) ;
#83548=EDGE_LOOP ( 'NONE', ( #28869, #92520 ) ) ;
#83591=COLOUR_RGB ( '', 0.72549020, 0.75294118, 0.79215686) ;
#83921=CARTESIAN_POINT ( 'NONE',  ( 2.897438467171757030E-16, 23.03999999999999915, 0.000000000000000000 ) ) ;
#84196=CARTESIAN_POINT ( 'NONE',  ( -7.598395483715266452E-32, -2.710505431213761085E-16, 0.000000000000000000 ) ) ;
#84199=CIRCLE ( 'NONE', #49074, 1.499999999999999112 ) ;
#84438=CARTESIAN_POINT ( 'NONE',  ( -2.999999999999999556, 21.83999999999999986, 0.000000000000000000 ) ) ;
#84532=VERTEX_POINT ( 'NONE', #84438 ) ;
#84644=AXIS2_PLACEMENT_3D ( 'NONE', #73328, #88340, #20835 ) ;
#84738=AXIS2_PLACEMENT_3D ( 'NONE', #27140, #34142, #41195 ) ;
#85048=LINE ( 'NONE', #77531, #2715 ) ;
#85072=ORIENTED_EDGE ( 'NONE', *, *, #56214, .F. ) ;
#85535=DIRECTION ( 'NONE',  ( 1.257568779154408793E-17, 1.000000000000000000, -0.000000000000000000 ) ) ;
#85832=ORIENTED_EDGE ( 'NONE', *, *, #68028, .T. ) ;
#86217=CIRCLE ( 'NONE', #84644, 5.999999999999998224 ) ;
#86449=FACE_OUTER_BOUND ( 'NONE', #96986, .T. ) ;
#86742=TOROIDAL_SURFACE ( 'NONE', #43605, 3.699999999999999289, 0.2999999999999999889 ) ;
#87044=CARTESIAN_POINT ( 'NONE',  ( 3.799999999999998934, 1.639999999999999014, 4.653657836759941744E-16 ) ) ;
#87086=DIRECTION ( 'NONE',  ( 1.257568779154408793E-17, 1.000000000000000000, -0.000000000000000000 ) ) ;
#87238=AXIS2_PLACEMENT_3D ( 'NONE', #64234, #74200, #95745 ) ;
#87334=VERTEX_POINT ( 'NONE', #76181 ) ;
#87377=CARTESIAN_POINT ( 'NONE',  ( -3.999999999999999112, 1.839999999999999636, 0.000000000000000000 ) ) ;
#87748=EDGE_LOOP ( 'NONE', ( #85072, #62904, #16487, #91788 ) ) ;
#88262=EDGE_CURVE ( 'NONE', #46930, #44781, #66473, .T. ) ;
#88330=AXIS2_PLACEMENT_3D ( 'NONE', #84196, #68692, #39185 ) ;
#88340=DIRECTION ( 'NONE',  ( -0.000000000000000000, 0.000000000000000000, -1.000000000000000000 ) ) ;
#88947=DIRECTION ( 'NONE',  ( -1.000000000000000000, 0.000000000000000000, 0.000000000000000000 ) ) ;
#89288=CARTESIAN_POINT ( 'NONE',  ( 2.062412797813223616E-17, 1.639999999999999014, 0.000000000000000000 ) ) ;
#89435=DIRECTION ( 'NONE',  ( -0.000000000000000000, 0.000000000000000000, -1.000000000000000000 ) ) ;
#89719=PRODUCT_CONTEXT ( 'NONE', #42329, 'mechanical' ) ;
#89907=VERTEX_POINT ( 'NONE', #11508 ) ;
#90172=AXIS2_PLACEMENT_3D ( 'NONE', #70344, #68869, #8356 ) ;
#90654=DIRECTION ( 'NONE',  ( 1.000000000000000000, 0.000000000000000000, 0.000000000000000000 ) ) ;
#90954=CYLINDRICAL_SURFACE ( 'NONE', #53796, 3.999999999999999112 ) ;
#91120=CIRCLE ( 'NONE', #12891, 3.000000000000000000 ) ;
#91788=ORIENTED_EDGE ( 'NONE', *, *, #82949, .F. ) ;
#91800=DIRECTION ( 'NONE',  ( 1.257568779154408793E-17, 1.000000000000000000, -0.000000000000000000 ) ) ;
#92331=DIRECTION ( 'NONE',  ( -1.000000000000000000, 0.000000000000000000, 0.000000000000000000 ) ) ;
#92394=CARTESIAN_POINT ( 'NONE',  ( 7.347880794884118750E-16, 17.03999999999999915, 0.000000000000000000 ) ) ;
#92520=ORIENTED_EDGE ( 'NONE', *, *, #25464, .T. ) ;
#92696=DIRECTION ( 'NONE',  ( -1.257568779154408793E-17, -1.000000000000000000, 0.000000000000000000 ) ) ;
#92794=FILL_AREA_STYLE_COLOUR ( '', #47055 ) ;
#93033=CIRCLE ( 'NONE', #19594, 0.2000000000000000944 ) ;
#93288=( LENGTH_UNIT ( ) NAMED_UNIT ( * ) SI_UNIT ( .MILLI., .METRE. ) );
#93361=ADVANCED_FACE ( 'NONE', ( #77471 ), #74047, .T. ) ;
#93381=( GEOMETRIC_REPRESENTATION_CONTEXT ( 3 ) GLOBAL_UNCERTAINTY_ASSIGNED_CONTEXT ( ( #4516 ) ) GLOBAL_UNIT_ASSIGNED_CONTEXT ( ( #93288, #24324, #32777 ) ) REPRESENTATION_CONTEXT ( 'NONE', 'WORKASPACE' ) );
#93792=( NAMED_UNIT ( * ) PLANE_ANGLE_UNIT ( ) SI_UNIT ( $, .RADIAN. ) );
#94145=VECTOR ( 'NONE', #22388, 1000.000000000000000 ) ;
#94402=COLOUR_RGB ( '', 0.09019608, 0.27058824, 0.51372549) ;
#94575=SURFACE_STYLE_FILL_AREA ( #41107 ) ;
#94809=EDGE_CURVE ( 'NONE', #87334, #62932, #62913, .T. ) ;
#94876=PLANE ( 'NONE',  #40967 ) ;
#95402=EDGE_CURVE ( 'NONE', #11994, #12652, #24674, .T. ) ;
#95745=DIRECTION ( 'NONE',  ( 1.000000000000000000, 0.000000000000000000, 0.000000000000000000 ) ) ;
#95802=AXIS2_PLACEMENT_3D ( 'NONE', #62299, #70818, #10794 ) ;
#95845=ORIENTED_EDGE ( 'NONE', *, *, #78802, .F. ) ;
#96380=DIRECTION ( 'NONE',  ( 1.000000000000000000, -1.257568779154408485E-17, 0.000000000000000000 ) ) ;
#96661=ADVANCED_FACE ( 'NONE', ( #30851 ), #64395, .T. ) ;
#96986=EDGE_LOOP ( 'NONE', ( #6634, #5880, #98828, #31625 ) ) ;
#97540=CIRCLE ( 'NONE', #54392, 1.499999999999998668 ) ;
#97559=DIRECTION ( 'NONE',  ( 1.257568779154408793E-17, 1.000000000000000000, -0.000000000000000000 ) ) ;
#97928=EDGE_CURVE ( 'NONE', #57215, #56371, #46997, .T. ) ;
#97951=DIRECTION ( 'NONE',  ( -1.000000000000000000, 0.000000000000000000, 0.000000000000000000 ) ) ;
#98193=VERTEX_POINT ( 'NONE', #65474 ) ;
#98447=DIRECTION ( 'NONE',  ( 1.257568779154408793E-17, 1.000000000000000000, -0.000000000000000000 ) ) ;
#98572=PRODUCT ( '1.4 Rivet', '1.4 Rivet', '', ( #89719 ) ) ;
#98772=EDGE_LOOP ( 'NONE', ( #73876, #58469, #32727, #5067 ) ) ;
#98825=EDGE_CURVE ( 'NONE', #62932, #56371, #75761, .T. ) ;
#98828=ORIENTED_EDGE ( 'NONE', *, *, #2099, .T. ) ;
#98967=COLOUR_RGB ( '', 0.66274510, 0.83137255, 0.94901961) ;
ENDSEC;
END-ISO-10303-21;
